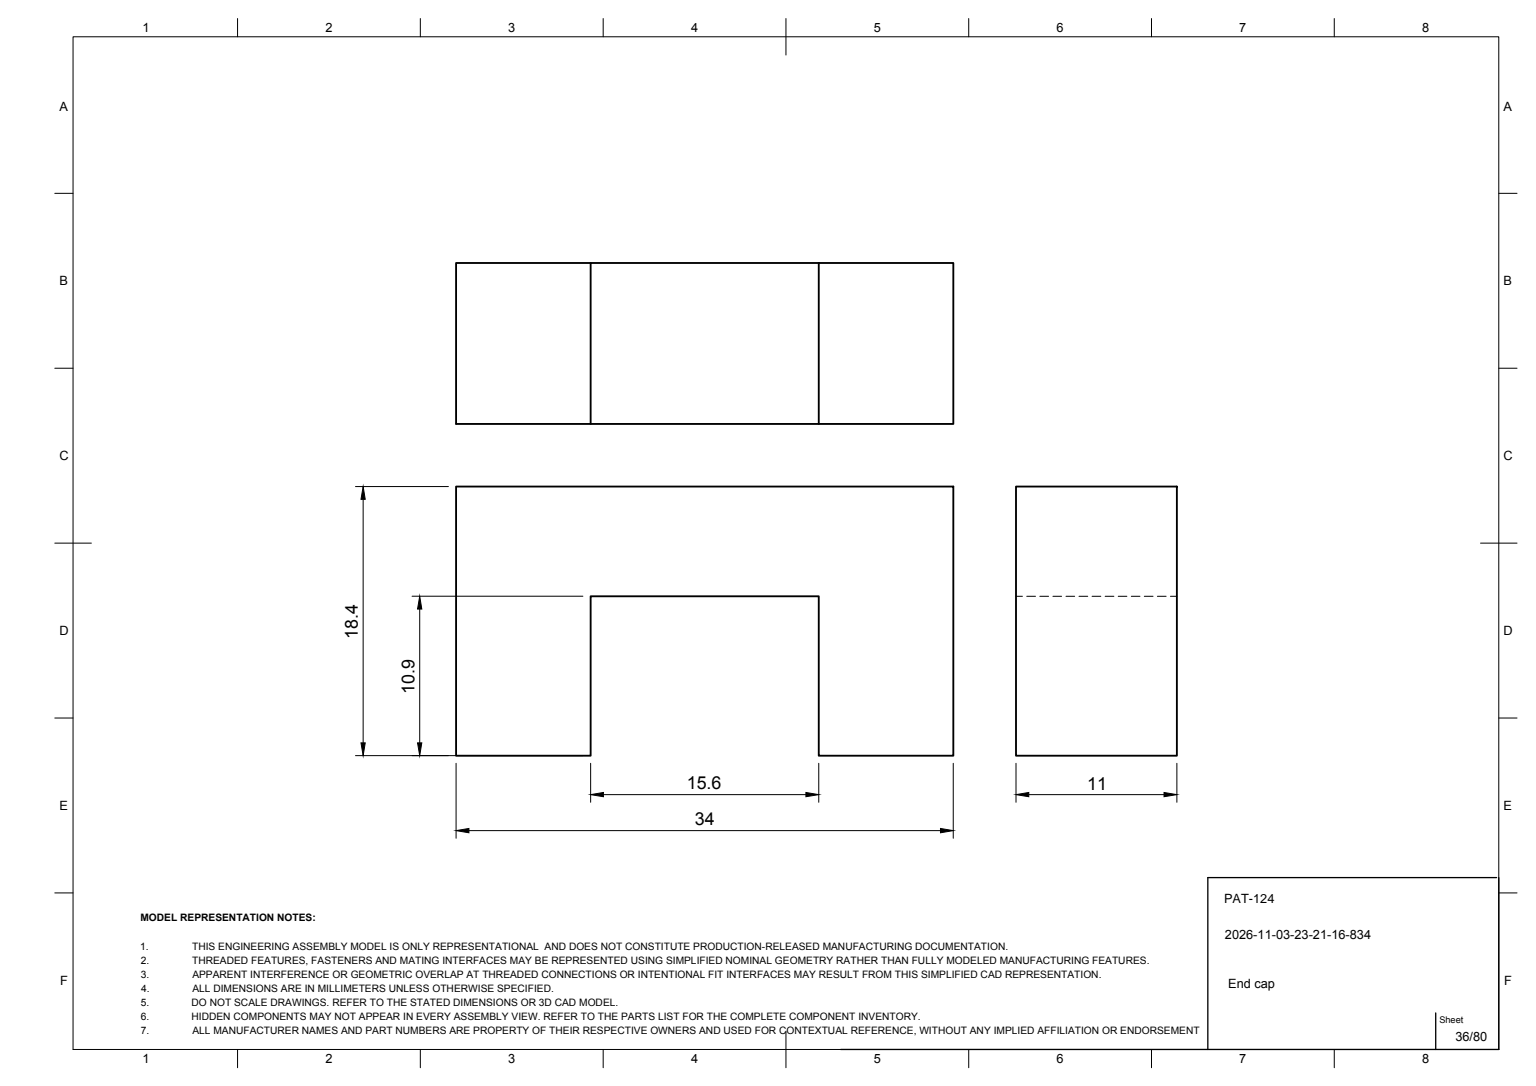
ISO-10303-21;
HEADER;
/* Generated by software containing ST-Developer
 * from STEP Tools, Inc. (www.steptools.com) 
 */

FILE_DESCRIPTION(
/* description */ ('XY cross-slide table'),
/* implementation_level */ '2;1');

FILE_NAME(
/* name */ 'End cap.step',
/* time_stamp */ '2026-10-28T03:22:46-07:00',
/* author */ (''),
/* organization */ (''),
/* preprocessor_version */ 'ST-DEVELOPER v20.2',
/* originating_system */ 'Autodesk Translation Framework v15.17.0.0',
/* authorisation */ '');

FILE_SCHEMA (('AUTOMOTIVE_DESIGN { 1 0 10303 214 3 1 1 }'));
ENDSEC;

DATA;
#10=MECHANICAL_DESIGN_GEOMETRIC_PRESENTATION_REPRESENTATION('',(#1711),#62984);
#1530=SHAPE_REPRESENTATION_RELATIONSHIP('SRR','None',#63382,#1613);
#1613=ADVANCED_BREP_SHAPE_REPRESENTATION('',(#1824),#62919);
#1711=STYLED_ITEM('',(#63926),#1824);
#1824=MANIFOLD_SOLID_BREP('Body1',#23005);
#2467=PLANE('',#24700);
#2468=PLANE('',#24701);
#2469=PLANE('',#24702);
#2470=PLANE('',#24703);
#2471=PLANE('',#24704);
#2472=PLANE('',#24705);
#2473=PLANE('',#24706);
#2474=PLANE('',#24707);
#2475=PLANE('',#24708);
#2476=PLANE('',#24709);
#3196=FACE_OUTER_BOUND('',#4669,.T.);
#3197=FACE_OUTER_BOUND('',#4670,.T.);
#3198=FACE_OUTER_BOUND('',#4671,.T.);
#3199=FACE_OUTER_BOUND('',#4672,.T.);
#3200=FACE_OUTER_BOUND('',#4673,.T.);
#3201=FACE_OUTER_BOUND('',#4674,.T.);
#3202=FACE_OUTER_BOUND('',#4675,.T.);
#3203=FACE_OUTER_BOUND('',#4676,.T.);
#3204=FACE_OUTER_BOUND('',#4677,.T.);
#3205=FACE_OUTER_BOUND('',#4678,.T.);
#4669=EDGE_LOOP('',(#16372,#16373,#16374,#16375));
#4670=EDGE_LOOP('',(#16376,#16377,#16378,#16379));
#4671=EDGE_LOOP('',(#16380,#16381,#16382,#16383));
#4672=EDGE_LOOP('',(#16384,#16385,#16386,#16387));
#4673=EDGE_LOOP('',(#16388,#16389,#16390,#16391));
#4674=EDGE_LOOP('',(#16392,#16393,#16394,#16395));
#4675=EDGE_LOOP('',(#16396,#16397,#16398,#16399));
#4676=EDGE_LOOP('',(#16400,#16401,#16402,#16403));
#4677=EDGE_LOOP('',(#16404,#16405,#16406,#16407,#16408,#16409,#16410,#16411));
#4678=EDGE_LOOP('',(#16412,#16413,#16414,#16415,#16416,#16417,#16418,#16419));
#6279=LINE('',#35114,#7766);
#6280=LINE('',#35116,#7767);
#6281=LINE('',#35118,#7768);
#6282=LINE('',#35119,#7769);
#6283=LINE('',#35122,#7770);
#6284=LINE('',#35124,#7771);
#6285=LINE('',#35125,#7772);
#6286=LINE('',#35128,#7773);
#6287=LINE('',#35130,#7774);
#6288=LINE('',#35131,#7775);
#6289=LINE('',#35134,#7776);
#6290=LINE('',#35136,#7777);
#6291=LINE('',#35137,#7778);
#6292=LINE('',#35140,#7779);
#6293=LINE('',#35142,#7780);
#6294=LINE('',#35143,#7781);
#6295=LINE('',#35146,#7782);
#6296=LINE('',#35148,#7783);
#6297=LINE('',#35149,#7784);
#6298=LINE('',#35152,#7785);
#6299=LINE('',#35154,#7786);
#6300=LINE('',#35155,#7787);
#6301=LINE('',#35157,#7788);
#6302=LINE('',#35158,#7789);
#7766=VECTOR('',#28236,1.);
#7767=VECTOR('',#28237,1.);
#7768=VECTOR('',#28238,1.);
#7769=VECTOR('',#28239,1.);
#7770=VECTOR('',#28242,1.);
#7771=VECTOR('',#28243,1.);
#7772=VECTOR('',#28244,1.);
#7773=VECTOR('',#28247,1.);
#7774=VECTOR('',#28248,1.);
#7775=VECTOR('',#28249,1.);
#7776=VECTOR('',#28252,1.);
#7777=VECTOR('',#28253,1.);
#7778=VECTOR('',#28254,1.);
#7779=VECTOR('',#28257,1.);
#7780=VECTOR('',#28258,1.);
#7781=VECTOR('',#28259,1.);
#7782=VECTOR('',#28262,1.);
#7783=VECTOR('',#28263,1.);
#7784=VECTOR('',#28264,1.);
#7785=VECTOR('',#28267,1.);
#7786=VECTOR('',#28268,1.);
#7787=VECTOR('',#28269,1.);
#7788=VECTOR('',#28272,1.);
#7789=VECTOR('',#28273,1.);
#10277=VERTEX_POINT('',#35112);
#10278=VERTEX_POINT('',#35113);
#10279=VERTEX_POINT('',#35115);
#10280=VERTEX_POINT('',#35117);
#10281=VERTEX_POINT('',#35121);
#10282=VERTEX_POINT('',#35123);
#10283=VERTEX_POINT('',#35127);
#10284=VERTEX_POINT('',#35129);
#10285=VERTEX_POINT('',#35133);
#10286=VERTEX_POINT('',#35135);
#10287=VERTEX_POINT('',#35139);
#10288=VERTEX_POINT('',#35141);
#10289=VERTEX_POINT('',#35145);
#10290=VERTEX_POINT('',#35147);
#10291=VERTEX_POINT('',#35151);
#10292=VERTEX_POINT('',#35153);
#12570=EDGE_CURVE('',#10277,#10278,#6279,.T.);
#12571=EDGE_CURVE('',#10277,#10279,#6280,.T.);
#12572=EDGE_CURVE('',#10280,#10279,#6281,.T.);
#12573=EDGE_CURVE('',#10278,#10280,#6282,.T.);
#12574=EDGE_CURVE('',#10278,#10281,#6283,.T.);
#12575=EDGE_CURVE('',#10282,#10280,#6284,.T.);
#12576=EDGE_CURVE('',#10281,#10282,#6285,.T.);
#12577=EDGE_CURVE('',#10281,#10283,#6286,.T.);
#12578=EDGE_CURVE('',#10284,#10282,#6287,.T.);
#12579=EDGE_CURVE('',#10283,#10284,#6288,.T.);
#12580=EDGE_CURVE('',#10283,#10285,#6289,.T.);
#12581=EDGE_CURVE('',#10286,#10284,#6290,.T.);
#12582=EDGE_CURVE('',#10285,#10286,#6291,.T.);
#12583=EDGE_CURVE('',#10285,#10287,#6292,.T.);
#12584=EDGE_CURVE('',#10288,#10286,#6293,.T.);
#12585=EDGE_CURVE('',#10287,#10288,#6294,.T.);
#12586=EDGE_CURVE('',#10287,#10289,#6295,.T.);
#12587=EDGE_CURVE('',#10290,#10288,#6296,.T.);
#12588=EDGE_CURVE('',#10289,#10290,#6297,.T.);
#12589=EDGE_CURVE('',#10289,#10291,#6298,.T.);
#12590=EDGE_CURVE('',#10292,#10290,#6299,.T.);
#12591=EDGE_CURVE('',#10291,#10292,#6300,.T.);
#12592=EDGE_CURVE('',#10291,#10277,#6301,.T.);
#12593=EDGE_CURVE('',#10279,#10292,#6302,.T.);
#16372=ORIENTED_EDGE('',*,*,#12570,.F.);
#16373=ORIENTED_EDGE('',*,*,#12571,.T.);
#16374=ORIENTED_EDGE('',*,*,#12572,.F.);
#16375=ORIENTED_EDGE('',*,*,#12573,.F.);
#16376=ORIENTED_EDGE('',*,*,#12574,.F.);
#16377=ORIENTED_EDGE('',*,*,#12573,.T.);
#16378=ORIENTED_EDGE('',*,*,#12575,.F.);
#16379=ORIENTED_EDGE('',*,*,#12576,.F.);
#16380=ORIENTED_EDGE('',*,*,#12577,.F.);
#16381=ORIENTED_EDGE('',*,*,#12576,.T.);
#16382=ORIENTED_EDGE('',*,*,#12578,.F.);
#16383=ORIENTED_EDGE('',*,*,#12579,.F.);
#16384=ORIENTED_EDGE('',*,*,#12580,.F.);
#16385=ORIENTED_EDGE('',*,*,#12579,.T.);
#16386=ORIENTED_EDGE('',*,*,#12581,.F.);
#16387=ORIENTED_EDGE('',*,*,#12582,.F.);
#16388=ORIENTED_EDGE('',*,*,#12583,.F.);
#16389=ORIENTED_EDGE('',*,*,#12582,.T.);
#16390=ORIENTED_EDGE('',*,*,#12584,.F.);
#16391=ORIENTED_EDGE('',*,*,#12585,.F.);
#16392=ORIENTED_EDGE('',*,*,#12586,.F.);
#16393=ORIENTED_EDGE('',*,*,#12585,.T.);
#16394=ORIENTED_EDGE('',*,*,#12587,.F.);
#16395=ORIENTED_EDGE('',*,*,#12588,.F.);
#16396=ORIENTED_EDGE('',*,*,#12589,.F.);
#16397=ORIENTED_EDGE('',*,*,#12588,.T.);
#16398=ORIENTED_EDGE('',*,*,#12590,.F.);
#16399=ORIENTED_EDGE('',*,*,#12591,.F.);
#16400=ORIENTED_EDGE('',*,*,#12592,.F.);
#16401=ORIENTED_EDGE('',*,*,#12591,.T.);
#16402=ORIENTED_EDGE('',*,*,#12593,.F.);
#16403=ORIENTED_EDGE('',*,*,#12571,.F.);
#16404=ORIENTED_EDGE('',*,*,#12592,.T.);
#16405=ORIENTED_EDGE('',*,*,#12570,.T.);
#16406=ORIENTED_EDGE('',*,*,#12574,.T.);
#16407=ORIENTED_EDGE('',*,*,#12577,.T.);
#16408=ORIENTED_EDGE('',*,*,#12580,.T.);
#16409=ORIENTED_EDGE('',*,*,#12583,.T.);
#16410=ORIENTED_EDGE('',*,*,#12586,.T.);
#16411=ORIENTED_EDGE('',*,*,#12589,.T.);
#16412=ORIENTED_EDGE('',*,*,#12593,.T.);
#16413=ORIENTED_EDGE('',*,*,#12590,.T.);
#16414=ORIENTED_EDGE('',*,*,#12587,.T.);
#16415=ORIENTED_EDGE('',*,*,#12584,.T.);
#16416=ORIENTED_EDGE('',*,*,#12581,.T.);
#16417=ORIENTED_EDGE('',*,*,#12578,.T.);
#16418=ORIENTED_EDGE('',*,*,#12575,.T.);
#16419=ORIENTED_EDGE('',*,*,#12572,.T.);
#21977=ADVANCED_FACE('',(#3196),#2467,.T.);
#21978=ADVANCED_FACE('',(#3197),#2468,.T.);
#21979=ADVANCED_FACE('',(#3198),#2469,.T.);
#21980=ADVANCED_FACE('',(#3199),#2470,.T.);
#21981=ADVANCED_FACE('',(#3200),#2471,.T.);
#21982=ADVANCED_FACE('',(#3201),#2472,.T.);
#21983=ADVANCED_FACE('',(#3202),#2473,.T.);
#21984=ADVANCED_FACE('',(#3203),#2474,.T.);
#21985=ADVANCED_FACE('',(#3204),#2475,.T.);
#21986=ADVANCED_FACE('',(#3205),#2476,.T.);
#23005=CLOSED_SHELL('',(#21977,#21978,#21979,#21980,#21981,#21982,#21983,
#21984,#21985,#21986));
#24699=AXIS2_PLACEMENT_3D('',#35110,#28232,#28233);
#24700=AXIS2_PLACEMENT_3D('',#35111,#28234,#28235);
#24701=AXIS2_PLACEMENT_3D('',#35120,#28240,#28241);
#24702=AXIS2_PLACEMENT_3D('',#35126,#28245,#28246);
#24703=AXIS2_PLACEMENT_3D('',#35132,#28250,#28251);
#24704=AXIS2_PLACEMENT_3D('',#35138,#28255,#28256);
#24705=AXIS2_PLACEMENT_3D('',#35144,#28260,#28261);
#24706=AXIS2_PLACEMENT_3D('',#35150,#28265,#28266);
#24707=AXIS2_PLACEMENT_3D('',#35156,#28270,#28271);
#24708=AXIS2_PLACEMENT_3D('',#35159,#28274,#28275);
#24709=AXIS2_PLACEMENT_3D('',#35160,#28276,#28277);
#28232=DIRECTION('axis',(0.,0.,1.));
#28233=DIRECTION('refdir',(1.,0.,0.));
#28234=DIRECTION('center_axis',(0.,0.,-1.));
#28235=DIRECTION('ref_axis',(0.,-1.,0.));
#28236=DIRECTION('',(0.,1.,0.));
#28237=DIRECTION('',(-1.,0.,0.));
#28238=DIRECTION('',(0.,-1.,0.));
#28239=DIRECTION('',(-1.,0.,0.));
#28240=DIRECTION('center_axis',(0.,1.,0.));
#28241=DIRECTION('ref_axis',(0.,0.,-1.));
#28242=DIRECTION('',(0.,0.,1.));
#28243=DIRECTION('',(0.,0.,-1.));
#28244=DIRECTION('',(-1.,0.,0.));
#28245=DIRECTION('center_axis',(0.,0.,-1.));
#28246=DIRECTION('ref_axis',(0.,-1.,0.));
#28247=DIRECTION('',(0.,1.,0.));
#28248=DIRECTION('',(0.,-1.,0.));
#28249=DIRECTION('',(-1.,0.,0.));
#28250=DIRECTION('center_axis',(0.,-1.,0.));
#28251=DIRECTION('ref_axis',(0.,0.,1.));
#28252=DIRECTION('',(0.,0.,-1.));
#28253=DIRECTION('',(0.,0.,1.));
#28254=DIRECTION('',(-1.,0.,0.));
#28255=DIRECTION('center_axis',(0.,0.,-1.));
#28256=DIRECTION('ref_axis',(0.,-1.,0.));
#28257=DIRECTION('',(0.,1.,0.));
#28258=DIRECTION('',(0.,-1.,0.));
#28259=DIRECTION('',(-1.,0.,0.));
#28260=DIRECTION('center_axis',(0.,1.,0.));
#28261=DIRECTION('ref_axis',(0.,0.,-1.));
#28262=DIRECTION('',(0.,0.,1.));
#28263=DIRECTION('',(0.,0.,-1.));
#28264=DIRECTION('',(-1.,0.,0.));
#28265=DIRECTION('center_axis',(0.,0.,1.));
#28266=DIRECTION('ref_axis',(0.,1.,0.));
#28267=DIRECTION('',(0.,-1.,0.));
#28268=DIRECTION('',(0.,1.,0.));
#28269=DIRECTION('',(-1.,0.,0.));
#28270=DIRECTION('center_axis',(0.,-1.,0.));
#28271=DIRECTION('ref_axis',(0.,0.,1.));
#28272=DIRECTION('',(0.,0.,-1.));
#28273=DIRECTION('',(0.,0.,1.));
#28274=DIRECTION('center_axis',(1.,0.,0.));
#28275=DIRECTION('ref_axis',(0.,0.,-1.));
#28276=DIRECTION('center_axis',(-1.,0.,0.));
#28277=DIRECTION('ref_axis',(0.,0.,1.));
#35110=CARTESIAN_POINT('',(0.,0.,0.));
#35111=CARTESIAN_POINT('Origin',(-1.97,-0.78,0.46));
#35112=CARTESIAN_POINT('',(-1.97,-1.7,0.46));
#35113=CARTESIAN_POINT('',(-1.97,-0.78,0.46));
#35114=CARTESIAN_POINT('',(-1.97,-1.7,0.46));
#35115=CARTESIAN_POINT('',(-3.07,-1.7,0.46));
#35116=CARTESIAN_POINT('',(-1.97,-1.7,0.46));
#35117=CARTESIAN_POINT('',(-3.07,-0.78,0.46));
#35118=CARTESIAN_POINT('',(-3.07,-1.7,0.46));
#35119=CARTESIAN_POINT('',(-1.97,-0.78,0.46));
#35120=CARTESIAN_POINT('Origin',(-1.97,-0.78,1.55));
#35121=CARTESIAN_POINT('',(-1.97,-0.78,1.55));
#35122=CARTESIAN_POINT('',(-1.97,-0.78,0.46));
#35123=CARTESIAN_POINT('',(-3.07,-0.78,1.55));
#35124=CARTESIAN_POINT('',(-3.07,-0.78,0.46));
#35125=CARTESIAN_POINT('',(-1.97,-0.78,1.55));
#35126=CARTESIAN_POINT('Origin',(-1.97,0.78,1.55));
#35127=CARTESIAN_POINT('',(-1.97,0.78,1.55));
#35128=CARTESIAN_POINT('',(-1.97,-0.78,1.55));
#35129=CARTESIAN_POINT('',(-3.07,0.78,1.55));
#35130=CARTESIAN_POINT('',(-3.07,-0.78,1.55));
#35131=CARTESIAN_POINT('',(-1.97,0.78,1.55));
#35132=CARTESIAN_POINT('Origin',(-1.97,0.78,0.46));
#35133=CARTESIAN_POINT('',(-1.97,0.78,0.46));
#35134=CARTESIAN_POINT('',(-1.97,0.78,1.55));
#35135=CARTESIAN_POINT('',(-3.07,0.78,0.46));
#35136=CARTESIAN_POINT('',(-3.07,0.78,1.55));
#35137=CARTESIAN_POINT('',(-1.97,0.78,0.46));
#35138=CARTESIAN_POINT('Origin',(-1.97,1.7,0.46));
#35139=CARTESIAN_POINT('',(-1.97,1.7,0.46));
#35140=CARTESIAN_POINT('',(-1.97,0.78,0.46));
#35141=CARTESIAN_POINT('',(-3.07,1.7,0.46));
#35142=CARTESIAN_POINT('',(-3.07,0.78,0.46));
#35143=CARTESIAN_POINT('',(-1.97,1.7,0.46));
#35144=CARTESIAN_POINT('Origin',(-1.97,1.7,2.3));
#35145=CARTESIAN_POINT('',(-1.97,1.7,2.3));
#35146=CARTESIAN_POINT('',(-1.97,1.7,0.46));
#35147=CARTESIAN_POINT('',(-3.07,1.7,2.3));
#35148=CARTESIAN_POINT('',(-3.07,1.7,0.46));
#35149=CARTESIAN_POINT('',(-1.97,1.7,2.3));
#35150=CARTESIAN_POINT('Origin',(-1.97,-1.7,2.3));
#35151=CARTESIAN_POINT('',(-1.97,-1.7,2.3));
#35152=CARTESIAN_POINT('',(-1.97,1.7,2.3));
#35153=CARTESIAN_POINT('',(-3.07,-1.7,2.3));
#35154=CARTESIAN_POINT('',(-3.07,1.7,2.3));
#35155=CARTESIAN_POINT('',(-1.97,-1.7,2.3));
#35156=CARTESIAN_POINT('Origin',(-1.97,-1.7,0.46));
#35157=CARTESIAN_POINT('',(-1.97,-1.7,2.3));
#35158=CARTESIAN_POINT('',(-3.07,-1.7,2.3));
#35159=CARTESIAN_POINT('Origin',(-1.97,0.,1.38));
#35160=CARTESIAN_POINT('Origin',(-3.07,0.,1.38));
#62820=UNCERTAINTY_MEASURE_WITH_UNIT(LENGTH_MEASURE(0.001),#62985,
'DISTANCE_ACCURACY_VALUE',
'Maximum model space distance between geometric entities at asserted c
onnectivities');
#62885=UNCERTAINTY_MEASURE_WITH_UNIT(LENGTH_MEASURE(0.001),#62985,
'DISTANCE_ACCURACY_VALUE',
'Maximum model space distance between geometric entities at asserted c
onnectivities');
#62919=(
GEOMETRIC_REPRESENTATION_CONTEXT(3)
GLOBAL_UNCERTAINTY_ASSIGNED_CONTEXT((#62820))
GLOBAL_UNIT_ASSIGNED_CONTEXT((#62985,#62987,#62988))
REPRESENTATION_CONTEXT('','3D')
);
#62984=(
GEOMETRIC_REPRESENTATION_CONTEXT(3)
GLOBAL_UNCERTAINTY_ASSIGNED_CONTEXT((#62885))
GLOBAL_UNIT_ASSIGNED_CONTEXT((#62985,#62987,#62988))
REPRESENTATION_CONTEXT('','3D')
);
#62985=(
LENGTH_UNIT()
NAMED_UNIT(*)
SI_UNIT(.CENTI.,.METRE.)
);
#62987=(
NAMED_UNIT(*)
PLANE_ANGLE_UNIT()
SI_UNIT($,.RADIAN.)
);
#62988=(
NAMED_UNIT(*)
SI_UNIT($,.STERADIAN.)
SOLID_ANGLE_UNIT()
);
#63022=SHAPE_DEFINITION_REPRESENTATION(#63130,#63382);
#63130=PRODUCT_DEFINITION_SHAPE('',$,#63481);
#63382=SHAPE_REPRESENTATION('',(#24699),#62919);
#63447=PRODUCT_DEFINITION_CONTEXT('part definition',#63743,'design');
#63481=PRODUCT_DEFINITION('End cap','End cap',#63579,#63447);
#63579=PRODUCT_DEFINITION_FORMATION('',$,#63778);
#63743=APPLICATION_CONTEXT(
'Core Data for Automotive Mechanical Design Process');
#63744=PRODUCT_CONTEXT('part definition',#63743,'mechanical');
#63778=PRODUCT('End cap','End cap','End cap',(#63744));
#63920=COLOUR_RGB('Off White',0.89,0.88,0.83);
#63921=FILL_AREA_STYLE_COLOUR('',#63920);
#63922=FILL_AREA_STYLE('',(#63921));
#63923=SURFACE_STYLE_FILL_AREA(#63922);
#63924=SURFACE_SIDE_STYLE('',(#63923));
#63925=SURFACE_STYLE_USAGE(.BOTH.,#63924);
#63926=PRESENTATION_STYLE_ASSIGNMENT((#63925));
ENDSEC;
END-ISO-10303-21;
